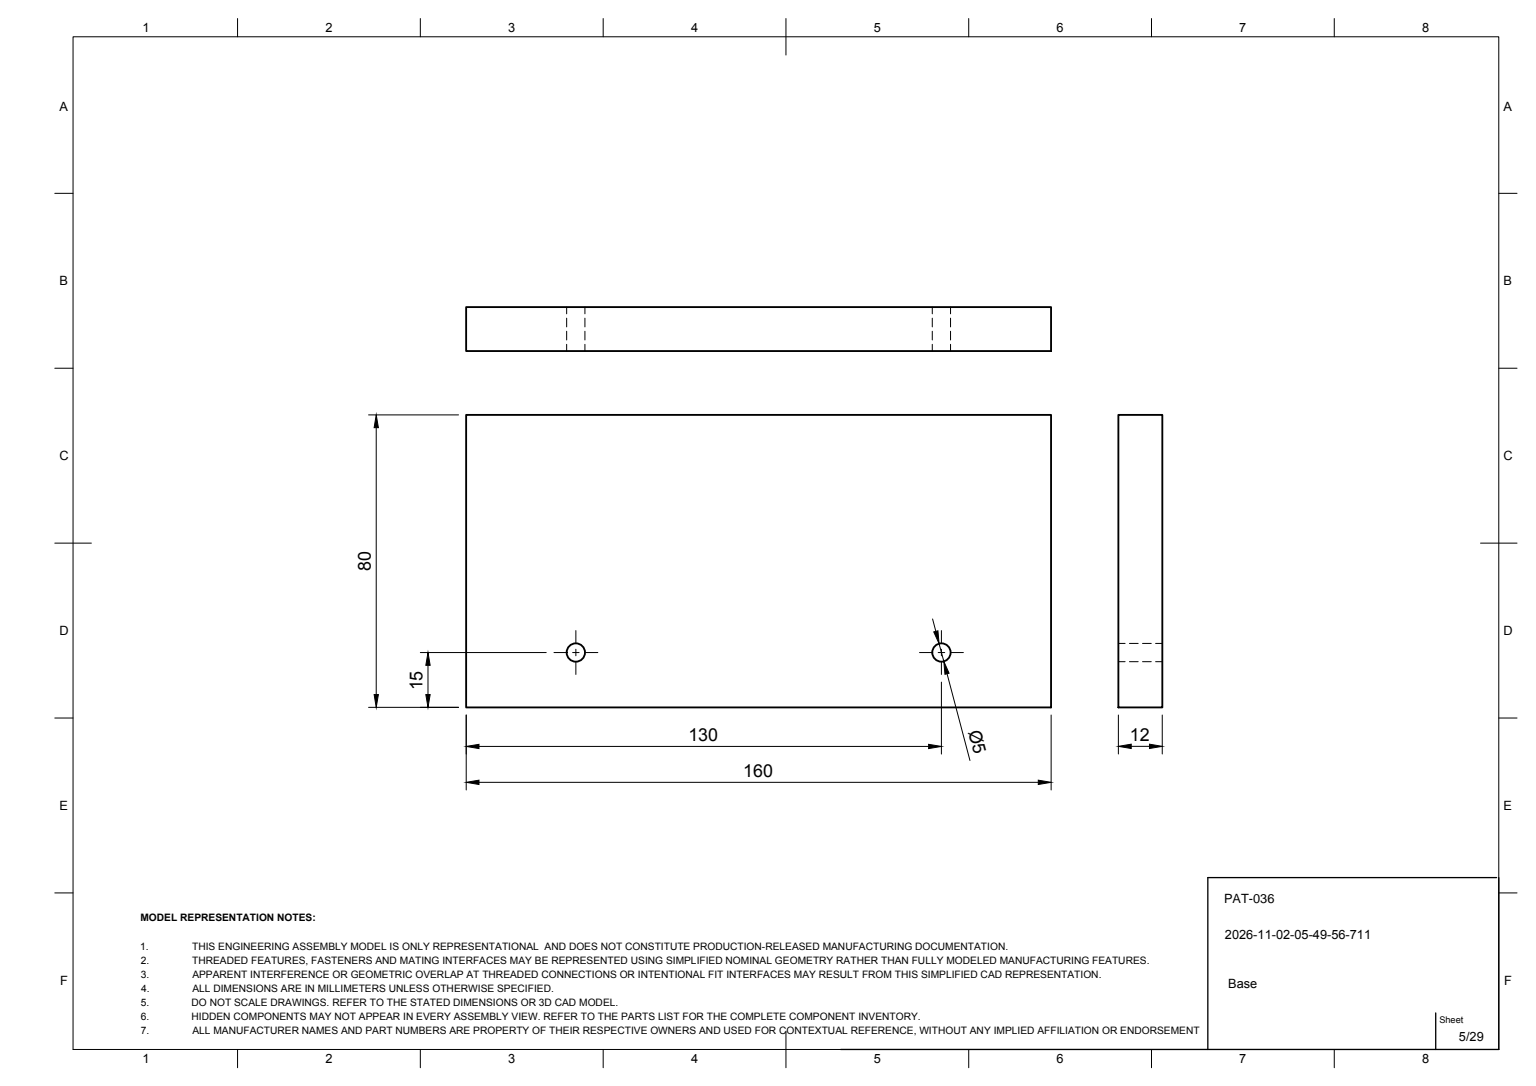
ISO-10303-21;
HEADER;
/* Generated by software containing ST-Developer
 * from STEP Tools, Inc. (www.steptools.com) 
 */

FILE_DESCRIPTION(
/* description */ ('Flange-mounted spindle'),
/* implementation_level */ '2;1');

FILE_NAME(
/* name */ 'Base.step',
/* time_stamp */ '2026-10-27T10:49:51-07:00',
/* author */ (''),
/* organization */ (''),
/* preprocessor_version */ 'ST-DEVELOPER v20.2',
/* originating_system */ 'Autodesk Translation Framework v15.17.0.0',
/* authorisation */ '');

FILE_SCHEMA (('AUTOMOTIVE_DESIGN { 1 0 10303 214 3 1 1 }'));
ENDSEC;

DATA;
#10=MECHANICAL_DESIGN_GEOMETRIC_PRESENTATION_REPRESENTATION('',(#338),#11764);
#284=SHAPE_REPRESENTATION_RELATIONSHIP('SRR','None',#11880,#311);
#311=ADVANCED_BREP_SHAPE_REPRESENTATION('',(#366),#11735);
#338=STYLED_ITEM('',(#12078),#366);
#366=MANIFOLD_SOLID_BREP('Body1',#6130);
#391=FACE_BOUND('',#1026,.T.);
#392=FACE_BOUND('',#1027,.T.);
#393=FACE_BOUND('',#1029,.T.);
#394=FACE_BOUND('',#1030,.T.);
#506=PLANE('',#6468);
#507=PLANE('',#6469);
#508=PLANE('',#6470);
#509=PLANE('',#6471);
#510=PLANE('',#6472);
#511=PLANE('',#6473);
#674=FACE_OUTER_BOUND('',#1019,.T.);
#675=FACE_OUTER_BOUND('',#1020,.T.);
#676=FACE_OUTER_BOUND('',#1021,.T.);
#677=FACE_OUTER_BOUND('',#1022,.T.);
#678=FACE_OUTER_BOUND('',#1023,.T.);
#679=FACE_OUTER_BOUND('',#1024,.T.);
#680=FACE_OUTER_BOUND('',#1025,.T.);
#681=FACE_OUTER_BOUND('',#1028,.T.);
#1019=EDGE_LOOP('',(#4005,#4006,#4007,#4008));
#1020=EDGE_LOOP('',(#4009,#4010,#4011,#4012));
#1021=EDGE_LOOP('',(#4013,#4014,#4015,#4016));
#1022=EDGE_LOOP('',(#4017,#4018,#4019,#4020));
#1023=EDGE_LOOP('',(#4021,#4022,#4023,#4024));
#1024=EDGE_LOOP('',(#4025,#4026,#4027,#4028));
#1025=EDGE_LOOP('',(#4029,#4030,#4031,#4032));
#1026=EDGE_LOOP('',(#4033));
#1027=EDGE_LOOP('',(#4034));
#1028=EDGE_LOOP('',(#4035,#4036,#4037,#4038));
#1029=EDGE_LOOP('',(#4039));
#1030=EDGE_LOOP('',(#4040));
#1479=LINE('',#9135,#1901);
#1480=LINE('',#9141,#1902);
#1481=LINE('',#9146,#1903);
#1482=LINE('',#9148,#1904);
#1483=LINE('',#9150,#1905);
#1484=LINE('',#9151,#1906);
#1485=LINE('',#9154,#1907);
#1486=LINE('',#9156,#1908);
#1487=LINE('',#9157,#1909);
#1488=LINE('',#9160,#1910);
#1489=LINE('',#9162,#1911);
#1490=LINE('',#9163,#1912);
#1491=LINE('',#9165,#1913);
#1492=LINE('',#9166,#1914);
#1901=VECTOR('',#7218,0.25);
#1902=VECTOR('',#7225,0.25);
#1903=VECTOR('',#7230,1.);
#1904=VECTOR('',#7231,1.);
#1905=VECTOR('',#7232,1.);
#1906=VECTOR('',#7233,1.);
#1907=VECTOR('',#7236,1.);
#1908=VECTOR('',#7237,1.);
#1909=VECTOR('',#7238,1.);
#1910=VECTOR('',#7241,1.);
#1911=VECTOR('',#7242,1.);
#1912=VECTOR('',#7243,1.);
#1913=VECTOR('',#7246,1.);
#1914=VECTOR('',#7247,1.);
#2323=CIRCLE('',#6463,0.25);
#2324=CIRCLE('',#6464,0.25);
#2325=CIRCLE('',#6466,0.25);
#2326=CIRCLE('',#6467,0.25);
#2649=VERTEX_POINT('',#9132);
#2650=VERTEX_POINT('',#9134);
#2651=VERTEX_POINT('',#9138);
#2652=VERTEX_POINT('',#9140);
#2653=VERTEX_POINT('',#9144);
#2654=VERTEX_POINT('',#9145);
#2655=VERTEX_POINT('',#9147);
#2656=VERTEX_POINT('',#9149);
#2657=VERTEX_POINT('',#9153);
#2658=VERTEX_POINT('',#9155);
#2659=VERTEX_POINT('',#9159);
#2660=VERTEX_POINT('',#9161);
#3195=EDGE_CURVE('',#2649,#2649,#2323,.T.);
#3196=EDGE_CURVE('',#2649,#2650,#1479,.T.);
#3197=EDGE_CURVE('',#2650,#2650,#2324,.T.);
#3198=EDGE_CURVE('',#2651,#2651,#2325,.T.);
#3199=EDGE_CURVE('',#2651,#2652,#1480,.T.);
#3200=EDGE_CURVE('',#2652,#2652,#2326,.T.);
#3201=EDGE_CURVE('',#2653,#2654,#1481,.T.);
#3202=EDGE_CURVE('',#2654,#2655,#1482,.T.);
#3203=EDGE_CURVE('',#2656,#2655,#1483,.T.);
#3204=EDGE_CURVE('',#2653,#2656,#1484,.T.);
#3205=EDGE_CURVE('',#2657,#2653,#1485,.T.);
#3206=EDGE_CURVE('',#2658,#2656,#1486,.T.);
#3207=EDGE_CURVE('',#2657,#2658,#1487,.T.);
#3208=EDGE_CURVE('',#2659,#2657,#1488,.T.);
#3209=EDGE_CURVE('',#2660,#2658,#1489,.T.);
#3210=EDGE_CURVE('',#2659,#2660,#1490,.T.);
#3211=EDGE_CURVE('',#2654,#2659,#1491,.T.);
#3212=EDGE_CURVE('',#2655,#2660,#1492,.T.);
#4005=ORIENTED_EDGE('',*,*,#3195,.F.);
#4006=ORIENTED_EDGE('',*,*,#3196,.T.);
#4007=ORIENTED_EDGE('',*,*,#3197,.F.);
#4008=ORIENTED_EDGE('',*,*,#3196,.F.);
#4009=ORIENTED_EDGE('',*,*,#3198,.F.);
#4010=ORIENTED_EDGE('',*,*,#3199,.T.);
#4011=ORIENTED_EDGE('',*,*,#3200,.F.);
#4012=ORIENTED_EDGE('',*,*,#3199,.F.);
#4013=ORIENTED_EDGE('',*,*,#3201,.T.);
#4014=ORIENTED_EDGE('',*,*,#3202,.T.);
#4015=ORIENTED_EDGE('',*,*,#3203,.F.);
#4016=ORIENTED_EDGE('',*,*,#3204,.F.);
#4017=ORIENTED_EDGE('',*,*,#3205,.T.);
#4018=ORIENTED_EDGE('',*,*,#3204,.T.);
#4019=ORIENTED_EDGE('',*,*,#3206,.F.);
#4020=ORIENTED_EDGE('',*,*,#3207,.F.);
#4021=ORIENTED_EDGE('',*,*,#3208,.T.);
#4022=ORIENTED_EDGE('',*,*,#3207,.T.);
#4023=ORIENTED_EDGE('',*,*,#3209,.F.);
#4024=ORIENTED_EDGE('',*,*,#3210,.F.);
#4025=ORIENTED_EDGE('',*,*,#3211,.T.);
#4026=ORIENTED_EDGE('',*,*,#3210,.T.);
#4027=ORIENTED_EDGE('',*,*,#3212,.F.);
#4028=ORIENTED_EDGE('',*,*,#3202,.F.);
#4029=ORIENTED_EDGE('',*,*,#3212,.T.);
#4030=ORIENTED_EDGE('',*,*,#3209,.T.);
#4031=ORIENTED_EDGE('',*,*,#3206,.T.);
#4032=ORIENTED_EDGE('',*,*,#3203,.T.);
#4033=ORIENTED_EDGE('',*,*,#3197,.T.);
#4034=ORIENTED_EDGE('',*,*,#3200,.T.);
#4035=ORIENTED_EDGE('',*,*,#3211,.F.);
#4036=ORIENTED_EDGE('',*,*,#3201,.F.);
#4037=ORIENTED_EDGE('',*,*,#3205,.F.);
#4038=ORIENTED_EDGE('',*,*,#3208,.F.);
#4039=ORIENTED_EDGE('',*,*,#3195,.T.);
#4040=ORIENTED_EDGE('',*,*,#3198,.T.);
#5625=CYLINDRICAL_SURFACE('',#6462,0.25);
#5626=CYLINDRICAL_SURFACE('',#6465,0.25);
#5785=ADVANCED_FACE('',(#674),#5625,.F.);
#5786=ADVANCED_FACE('',(#675),#5626,.F.);
#5787=ADVANCED_FACE('',(#676),#506,.T.);
#5788=ADVANCED_FACE('',(#677),#507,.T.);
#5789=ADVANCED_FACE('',(#678),#508,.T.);
#5790=ADVANCED_FACE('',(#679),#509,.T.);
#5791=ADVANCED_FACE('',(#680,#391,#392),#510,.T.);
#5792=ADVANCED_FACE('',(#681,#393,#394),#511,.F.);
#6130=CLOSED_SHELL('',(#5785,#5786,#5787,#5788,#5789,#5790,#5791,#5792));
#6461=AXIS2_PLACEMENT_3D('',#9130,#7212,#7213);
#6462=AXIS2_PLACEMENT_3D('',#9131,#7214,#7215);
#6463=AXIS2_PLACEMENT_3D('',#9133,#7216,#7217);
#6464=AXIS2_PLACEMENT_3D('',#9136,#7219,#7220);
#6465=AXIS2_PLACEMENT_3D('',#9137,#7221,#7222);
#6466=AXIS2_PLACEMENT_3D('',#9139,#7223,#7224);
#6467=AXIS2_PLACEMENT_3D('',#9142,#7226,#7227);
#6468=AXIS2_PLACEMENT_3D('',#9143,#7228,#7229);
#6469=AXIS2_PLACEMENT_3D('',#9152,#7234,#7235);
#6470=AXIS2_PLACEMENT_3D('',#9158,#7239,#7240);
#6471=AXIS2_PLACEMENT_3D('',#9164,#7244,#7245);
#6472=AXIS2_PLACEMENT_3D('',#9167,#7248,#7249);
#6473=AXIS2_PLACEMENT_3D('',#9168,#7250,#7251);
#7212=DIRECTION('axis',(0.,0.,1.));
#7213=DIRECTION('refdir',(1.,0.,0.));
#7214=DIRECTION('center_axis',(0.,0.,1.));
#7215=DIRECTION('ref_axis',(1.,0.,0.));
#7216=DIRECTION('center_axis',(0.,0.,1.));
#7217=DIRECTION('ref_axis',(1.,0.,0.));
#7218=DIRECTION('',(0.,0.,1.));
#7219=DIRECTION('center_axis',(0.,0.,-1.));
#7220=DIRECTION('ref_axis',(1.,0.,0.));
#7221=DIRECTION('center_axis',(0.,0.,1.));
#7222=DIRECTION('ref_axis',(1.,0.,0.));
#7223=DIRECTION('center_axis',(0.,0.,1.));
#7224=DIRECTION('ref_axis',(1.,0.,0.));
#7225=DIRECTION('',(0.,0.,1.));
#7226=DIRECTION('center_axis',(0.,0.,-1.));
#7227=DIRECTION('ref_axis',(1.,0.,0.));
#7228=DIRECTION('center_axis',(0.,1.,0.));
#7229=DIRECTION('ref_axis',(-1.,0.,0.));
#7230=DIRECTION('',(-1.,0.,0.));
#7231=DIRECTION('',(0.,0.,1.));
#7232=DIRECTION('',(-1.,0.,0.));
#7233=DIRECTION('',(0.,0.,1.));
#7234=DIRECTION('center_axis',(1.,0.,0.));
#7235=DIRECTION('ref_axis',(0.,1.,0.));
#7236=DIRECTION('',(0.,1.,0.));
#7237=DIRECTION('',(0.,1.,0.));
#7238=DIRECTION('',(0.,0.,1.));
#7239=DIRECTION('center_axis',(0.,-1.,0.));
#7240=DIRECTION('ref_axis',(1.,0.,0.));
#7241=DIRECTION('',(1.,0.,0.));
#7242=DIRECTION('',(1.,0.,0.));
#7243=DIRECTION('',(0.,0.,1.));
#7244=DIRECTION('center_axis',(-1.,0.,0.));
#7245=DIRECTION('ref_axis',(0.,-1.,0.));
#7246=DIRECTION('',(0.,-1.,0.));
#7247=DIRECTION('',(0.,-1.,0.));
#7248=DIRECTION('center_axis',(0.,0.,1.));
#7249=DIRECTION('ref_axis',(1.,0.,0.));
#7250=DIRECTION('center_axis',(0.,0.,1.));
#7251=DIRECTION('ref_axis',(1.,0.,0.));
#9130=CARTESIAN_POINT('',(0.,0.,0.));
#9131=CARTESIAN_POINT('Origin',(-5.,-2.5,-0.1));
#9132=CARTESIAN_POINT('',(-5.25,-2.5,0.));
#9133=CARTESIAN_POINT('Origin',(-5.,-2.5,0.));
#9134=CARTESIAN_POINT('',(-5.25,-2.5,1.2));
#9135=CARTESIAN_POINT('',(-5.25,-2.5,-0.1));
#9136=CARTESIAN_POINT('Origin',(-5.,-2.5,1.2));
#9137=CARTESIAN_POINT('Origin',(5.,-2.5,-0.1));
#9138=CARTESIAN_POINT('',(4.75,-2.5,0.));
#9139=CARTESIAN_POINT('Origin',(5.,-2.5,0.));
#9140=CARTESIAN_POINT('',(4.75,-2.5,1.2));
#9141=CARTESIAN_POINT('',(4.75,-2.5,-0.1));
#9142=CARTESIAN_POINT('Origin',(5.,-2.5,1.2));
#9143=CARTESIAN_POINT('Origin',(8.,4.,0.));
#9144=CARTESIAN_POINT('',(8.,4.,0.));
#9145=CARTESIAN_POINT('',(-8.,4.,0.));
#9146=CARTESIAN_POINT('',(8.,4.,0.));
#9147=CARTESIAN_POINT('',(-8.,4.,1.2));
#9148=CARTESIAN_POINT('',(-8.,4.,0.));
#9149=CARTESIAN_POINT('',(8.,4.,1.2));
#9150=CARTESIAN_POINT('',(8.,4.,1.2));
#9151=CARTESIAN_POINT('',(8.,4.,0.));
#9152=CARTESIAN_POINT('Origin',(8.,-4.,0.));
#9153=CARTESIAN_POINT('',(8.,-4.,0.));
#9154=CARTESIAN_POINT('',(8.,-4.,0.));
#9155=CARTESIAN_POINT('',(8.,-4.,1.2));
#9156=CARTESIAN_POINT('',(8.,-4.,1.2));
#9157=CARTESIAN_POINT('',(8.,-4.,0.));
#9158=CARTESIAN_POINT('Origin',(-8.,-4.,0.));
#9159=CARTESIAN_POINT('',(-8.,-4.,0.));
#9160=CARTESIAN_POINT('',(-8.,-4.,0.));
#9161=CARTESIAN_POINT('',(-8.,-4.,1.2));
#9162=CARTESIAN_POINT('',(-8.,-4.,1.2));
#9163=CARTESIAN_POINT('',(-8.,-4.,0.));
#9164=CARTESIAN_POINT('Origin',(-8.,4.,0.));
#9165=CARTESIAN_POINT('',(-8.,4.,0.));
#9166=CARTESIAN_POINT('',(-8.,4.,1.2));
#9167=CARTESIAN_POINT('Origin',(0.,0.,1.2));
#9168=CARTESIAN_POINT('Origin',(0.,0.,0.));
#11703=UNCERTAINTY_MEASURE_WITH_UNIT(LENGTH_MEASURE(0.001),#11765,
'DISTANCE_ACCURACY_VALUE',
'Maximum model space distance between geometric entities at asserted c
onnectivities');
#11732=UNCERTAINTY_MEASURE_WITH_UNIT(LENGTH_MEASURE(0.001),#11765,
'DISTANCE_ACCURACY_VALUE',
'Maximum model space distance between geometric entities at asserted c
onnectivities');
#11735=(
GEOMETRIC_REPRESENTATION_CONTEXT(3)
GLOBAL_UNCERTAINTY_ASSIGNED_CONTEXT((#11703))
GLOBAL_UNIT_ASSIGNED_CONTEXT((#11765,#11767,#11768))
REPRESENTATION_CONTEXT('','3D')
);
#11764=(
GEOMETRIC_REPRESENTATION_CONTEXT(3)
GLOBAL_UNCERTAINTY_ASSIGNED_CONTEXT((#11732))
GLOBAL_UNIT_ASSIGNED_CONTEXT((#11765,#11767,#11768))
REPRESENTATION_CONTEXT('','3D')
);
#11765=(
LENGTH_UNIT()
NAMED_UNIT(*)
SI_UNIT(.CENTI.,.METRE.)
);
#11767=(
NAMED_UNIT(*)
PLANE_ANGLE_UNIT()
SI_UNIT($,.RADIAN.)
);
#11768=(
NAMED_UNIT(*)
SI_UNIT($,.STERADIAN.)
SOLID_ANGLE_UNIT()
);
#11771=SHAPE_DEFINITION_REPRESENTATION(#11802,#11880);
#11802=PRODUCT_DEFINITION_SHAPE('',$,#11912);
#11880=SHAPE_REPRESENTATION('',(#6461),#11735);
#11909=PRODUCT_DEFINITION_CONTEXT('part definition',#12004,'design');
#11912=PRODUCT_DEFINITION('Base','Base',#11943,#11909);
#11943=PRODUCT_DEFINITION_FORMATION('',$,#12008);
#12004=APPLICATION_CONTEXT(
'Core Data for Automotive Mechanical Design Process');
#12005=PRODUCT_CONTEXT('part definition',#12004,'mechanical');
#12008=PRODUCT('Base','Base','Base',(#12005));
#12072=COLOUR_RGB('Dark Blue',0.08,0.2,0.34);
#12073=FILL_AREA_STYLE_COLOUR('',#12072);
#12074=FILL_AREA_STYLE('',(#12073));
#12075=SURFACE_STYLE_FILL_AREA(#12074);
#12076=SURFACE_SIDE_STYLE('',(#12075));
#12077=SURFACE_STYLE_USAGE(.BOTH.,#12076);
#12078=PRESENTATION_STYLE_ASSIGNMENT((#12077));
ENDSEC;
END-ISO-10303-21;
